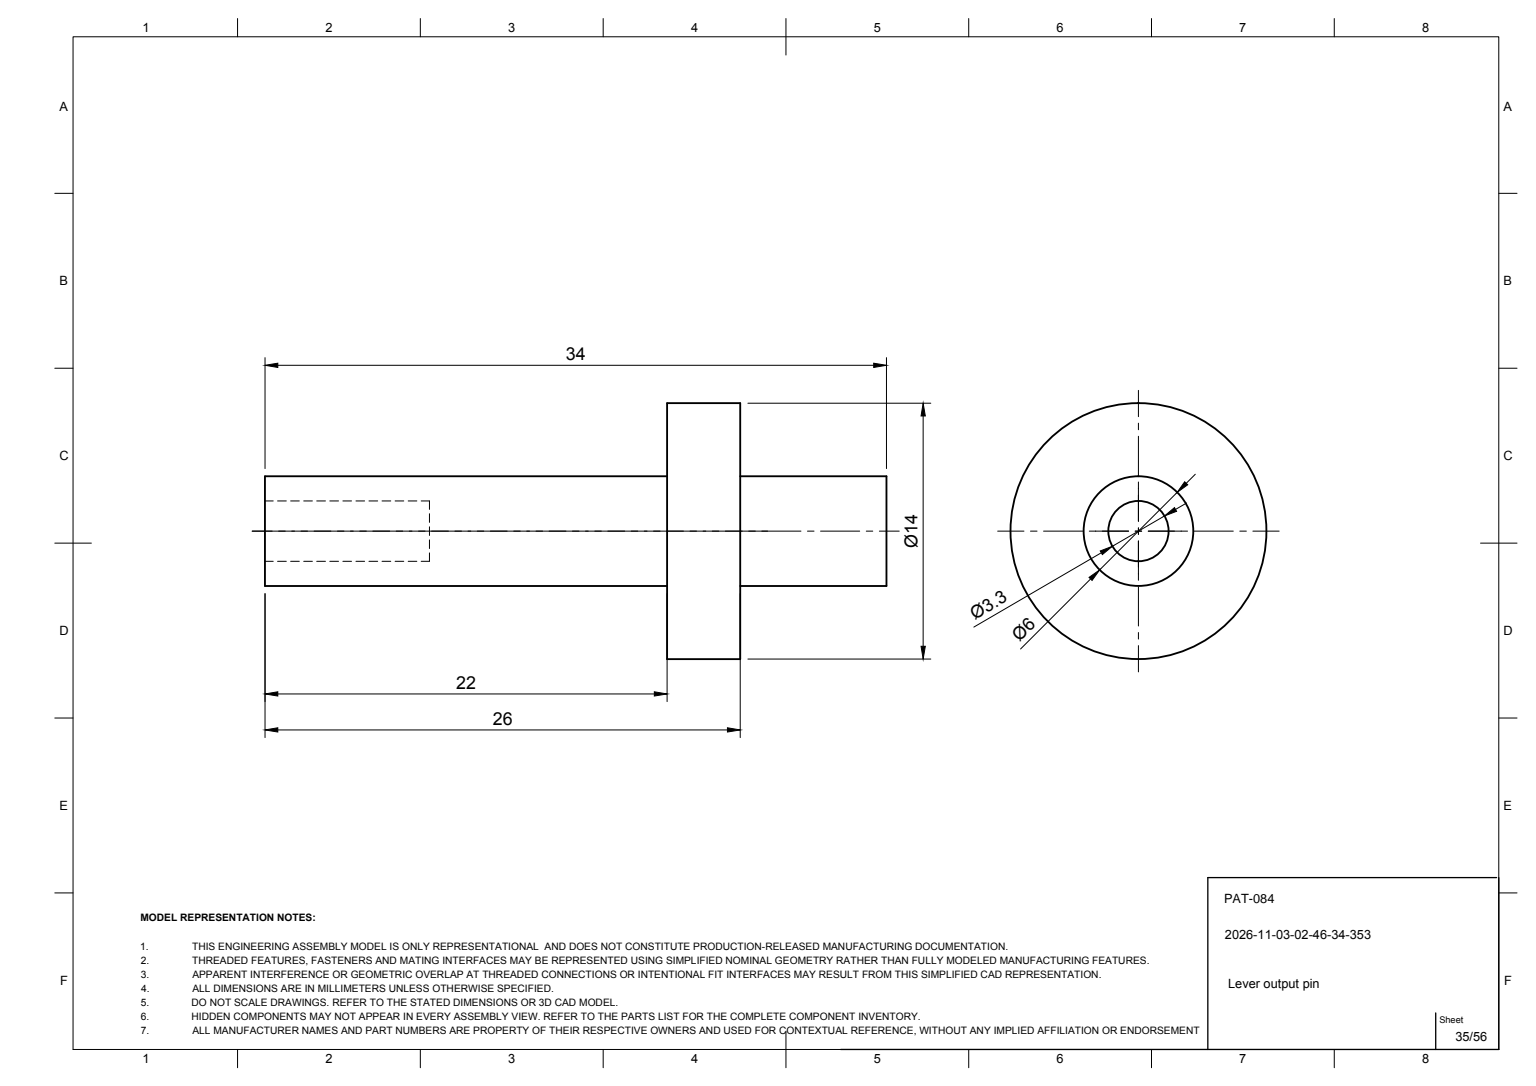
ISO-10303-21;
HEADER;
/* Generated by software containing ST-Developer
 * from STEP Tools, Inc. (www.steptools.com) 
 */

FILE_DESCRIPTION(
/* description */ ('Quick-return (Whitworth) mechanism'),
/* implementation_level */ '2;1');

FILE_NAME(
/* name */ 'Lever output pin.step',
/* time_stamp */ '2026-10-28T03:25:57-07:00',
/* author */ (''),
/* organization */ (''),
/* preprocessor_version */ 'ST-DEVELOPER v20.2',
/* originating_system */ 'Autodesk Translation Framework v15.17.0.0',
/* authorisation */ '');

FILE_SCHEMA (('AUTOMOTIVE_DESIGN { 1 0 10303 214 3 1 1 }'));
ENDSEC;

DATA;
#10=MECHANICAL_DESIGN_GEOMETRIC_PRESENTATION_REPRESENTATION('',(#523),#14878);
#427=SHAPE_REPRESENTATION_RELATIONSHIP('SRR','None',#15098,#471);
#471=ADVANCED_BREP_SHAPE_REPRESENTATION('',(#574),#14855);
#523=STYLED_ITEM('',(#15406),#574);
#574=MANIFOLD_SOLID_BREP('Body1',#7878);
#737=FACE_BOUND('',#1959,.T.);
#738=FACE_BOUND('',#1961,.T.);
#739=FACE_BOUND('',#1966,.T.);
#928=PLANE('',#9034);
#929=PLANE('',#9035);
#930=PLANE('',#9038);
#931=PLANE('',#9046);
#932=PLANE('',#9047);
#1344=FACE_OUTER_BOUND('',#1956,.T.);
#1345=FACE_OUTER_BOUND('',#1957,.T.);
#1346=FACE_OUTER_BOUND('',#1958,.T.);
#1347=FACE_OUTER_BOUND('',#1960,.T.);
#1348=FACE_OUTER_BOUND('',#1962,.T.);
#1349=FACE_OUTER_BOUND('',#1963,.T.);
#1350=FACE_OUTER_BOUND('',#1964,.T.);
#1351=FACE_OUTER_BOUND('',#1965,.T.);
#1352=FACE_OUTER_BOUND('',#1967,.T.);
#1956=EDGE_LOOP('',(#6492,#6493,#6494,#6495));
#1957=EDGE_LOOP('',(#6496));
#1958=EDGE_LOOP('',(#6497));
#1959=EDGE_LOOP('',(#6498));
#1960=EDGE_LOOP('',(#6499));
#1961=EDGE_LOOP('',(#6500));
#1962=EDGE_LOOP('',(#6501,#6502,#6503,#6504));
#1963=EDGE_LOOP('',(#6505,#6506,#6507,#6508));
#1964=EDGE_LOOP('',(#6509,#6510,#6511,#6512));
#1965=EDGE_LOOP('',(#6513));
#1966=EDGE_LOOP('',(#6514));
#1967=EDGE_LOOP('',(#6515));
#2435=LINE('',#13914,#2958);
#2436=LINE('',#13928,#2959);
#2437=LINE('',#13931,#2960);
#2438=LINE('',#13936,#2961);
#2958=VECTOR('',#10960,0.165);
#2959=VECTOR('',#10979,0.7);
#2960=VECTOR('',#10982,0.3);
#2961=VECTOR('',#10989,0.3);
#3530=CIRCLE('',#9032,0.165);
#3531=CIRCLE('',#9033,0.165);
#3532=CIRCLE('',#9036,0.7);
#3533=CIRCLE('',#9037,0.3);
#3534=CIRCLE('',#9039,0.7);
#3535=CIRCLE('',#9040,0.3);
#3536=CIRCLE('',#9043,0.3);
#3537=CIRCLE('',#9045,0.3);
#4051=VERTEX_POINT('',#13911);
#4052=VERTEX_POINT('',#13913);
#4053=VERTEX_POINT('',#13918);
#4054=VERTEX_POINT('',#13920);
#4055=VERTEX_POINT('',#13923);
#4056=VERTEX_POINT('',#13925);
#4057=VERTEX_POINT('',#13930);
#4058=VERTEX_POINT('',#13934);
#4903=EDGE_CURVE('',#4051,#4051,#3530,.T.);
#4904=EDGE_CURVE('',#4051,#4052,#2435,.T.);
#4905=EDGE_CURVE('',#4052,#4052,#3531,.T.);
#4906=EDGE_CURVE('',#4053,#4053,#3532,.T.);
#4907=EDGE_CURVE('',#4054,#4054,#3533,.T.);
#4908=EDGE_CURVE('',#4055,#4055,#3534,.T.);
#4909=EDGE_CURVE('',#4056,#4056,#3535,.T.);
#4910=EDGE_CURVE('',#4053,#4055,#2436,.T.);
#4911=EDGE_CURVE('',#4056,#4057,#2437,.T.);
#4912=EDGE_CURVE('',#4057,#4057,#3536,.T.);
#4913=EDGE_CURVE('',#4058,#4058,#3537,.T.);
#4914=EDGE_CURVE('',#4058,#4054,#2438,.T.);
#6492=ORIENTED_EDGE('',*,*,#4903,.F.);
#6493=ORIENTED_EDGE('',*,*,#4904,.T.);
#6494=ORIENTED_EDGE('',*,*,#4905,.F.);
#6495=ORIENTED_EDGE('',*,*,#4904,.F.);
#6496=ORIENTED_EDGE('',*,*,#4903,.T.);
#6497=ORIENTED_EDGE('',*,*,#4906,.T.);
#6498=ORIENTED_EDGE('',*,*,#4907,.F.);
#6499=ORIENTED_EDGE('',*,*,#4908,.F.);
#6500=ORIENTED_EDGE('',*,*,#4909,.F.);
#6501=ORIENTED_EDGE('',*,*,#4906,.F.);
#6502=ORIENTED_EDGE('',*,*,#4910,.T.);
#6503=ORIENTED_EDGE('',*,*,#4908,.T.);
#6504=ORIENTED_EDGE('',*,*,#4910,.F.);
#6505=ORIENTED_EDGE('',*,*,#4909,.T.);
#6506=ORIENTED_EDGE('',*,*,#4911,.T.);
#6507=ORIENTED_EDGE('',*,*,#4912,.T.);
#6508=ORIENTED_EDGE('',*,*,#4911,.F.);
#6509=ORIENTED_EDGE('',*,*,#4913,.F.);
#6510=ORIENTED_EDGE('',*,*,#4914,.T.);
#6511=ORIENTED_EDGE('',*,*,#4907,.T.);
#6512=ORIENTED_EDGE('',*,*,#4914,.F.);
#6513=ORIENTED_EDGE('',*,*,#4913,.T.);
#6514=ORIENTED_EDGE('',*,*,#4905,.T.);
#6515=ORIENTED_EDGE('',*,*,#4912,.F.);
#7335=CYLINDRICAL_SURFACE('',#9031,0.165);
#7336=CYLINDRICAL_SURFACE('',#9041,0.7);
#7337=CYLINDRICAL_SURFACE('',#9042,0.3);
#7338=CYLINDRICAL_SURFACE('',#9044,0.3);
#7675=ADVANCED_FACE('',(#1344),#7335,.F.);
#7676=ADVANCED_FACE('',(#1345),#928,.T.);
#7677=ADVANCED_FACE('',(#1346,#737),#929,.T.);
#7678=ADVANCED_FACE('',(#1347,#738),#930,.F.);
#7679=ADVANCED_FACE('',(#1348),#7336,.T.);
#7680=ADVANCED_FACE('',(#1349),#7337,.T.);
#7681=ADVANCED_FACE('',(#1350),#7338,.T.);
#7682=ADVANCED_FACE('',(#1351,#739),#931,.T.);
#7683=ADVANCED_FACE('',(#1352),#932,.F.);
#7878=CLOSED_SHELL('',(#7675,#7676,#7677,#7678,#7679,#7680,#7681,#7682,
#7683));
#9030=AXIS2_PLACEMENT_3D('',#13909,#10954,#10955);
#9031=AXIS2_PLACEMENT_3D('',#13910,#10956,#10957);
#9032=AXIS2_PLACEMENT_3D('',#13912,#10958,#10959);
#9033=AXIS2_PLACEMENT_3D('',#13915,#10961,#10962);
#9034=AXIS2_PLACEMENT_3D('',#13916,#10963,#10964);
#9035=AXIS2_PLACEMENT_3D('',#13917,#10965,#10966);
#9036=AXIS2_PLACEMENT_3D('',#13919,#10967,#10968);
#9037=AXIS2_PLACEMENT_3D('',#13921,#10969,#10970);
#9038=AXIS2_PLACEMENT_3D('',#13922,#10971,#10972);
#9039=AXIS2_PLACEMENT_3D('',#13924,#10973,#10974);
#9040=AXIS2_PLACEMENT_3D('',#13926,#10975,#10976);
#9041=AXIS2_PLACEMENT_3D('',#13927,#10977,#10978);
#9042=AXIS2_PLACEMENT_3D('',#13929,#10980,#10981);
#9043=AXIS2_PLACEMENT_3D('',#13932,#10983,#10984);
#9044=AXIS2_PLACEMENT_3D('',#13933,#10985,#10986);
#9045=AXIS2_PLACEMENT_3D('',#13935,#10987,#10988);
#9046=AXIS2_PLACEMENT_3D('',#13937,#10990,#10991);
#9047=AXIS2_PLACEMENT_3D('',#13938,#10992,#10993);
#10954=DIRECTION('axis',(0.,0.,1.));
#10955=DIRECTION('refdir',(1.,0.,0.));
#10956=DIRECTION('center_axis',(0.,0.,1.));
#10957=DIRECTION('ref_axis',(1.,0.,0.));
#10958=DIRECTION('center_axis',(0.,0.,1.));
#10959=DIRECTION('ref_axis',(1.,0.,0.));
#10960=DIRECTION('',(0.,0.,1.));
#10961=DIRECTION('center_axis',(0.,0.,-1.));
#10962=DIRECTION('ref_axis',(1.,0.,0.));
#10963=DIRECTION('center_axis',(0.,0.,1.));
#10964=DIRECTION('ref_axis',(1.,0.,0.));
#10965=DIRECTION('center_axis',(0.,0.,1.));
#10966=DIRECTION('ref_axis',(1.,0.,0.));
#10967=DIRECTION('center_axis',(0.,0.,1.));
#10968=DIRECTION('ref_axis',(1.,0.,0.));
#10969=DIRECTION('center_axis',(0.,0.,1.));
#10970=DIRECTION('ref_axis',(1.,0.,0.));
#10971=DIRECTION('center_axis',(0.,0.,1.));
#10972=DIRECTION('ref_axis',(1.,0.,0.));
#10973=DIRECTION('center_axis',(0.,0.,1.));
#10974=DIRECTION('ref_axis',(1.,0.,0.));
#10975=DIRECTION('center_axis',(0.,0.,-1.));
#10976=DIRECTION('ref_axis',(1.,0.,0.));
#10977=DIRECTION('center_axis',(0.,0.,1.));
#10978=DIRECTION('ref_axis',(1.,0.,0.));
#10979=DIRECTION('',(0.,0.,-1.));
#10980=DIRECTION('center_axis',(0.,0.,1.));
#10981=DIRECTION('ref_axis',(1.,0.,0.));
#10982=DIRECTION('',(0.,0.,-1.));
#10983=DIRECTION('center_axis',(0.,0.,1.));
#10984=DIRECTION('ref_axis',(1.,0.,0.));
#10985=DIRECTION('center_axis',(0.,0.,1.));
#10986=DIRECTION('ref_axis',(1.,0.,0.));
#10987=DIRECTION('center_axis',(0.,0.,1.));
#10988=DIRECTION('ref_axis',(1.,0.,0.));
#10989=DIRECTION('',(0.,0.,-1.));
#10990=DIRECTION('center_axis',(0.,0.,1.));
#10991=DIRECTION('ref_axis',(1.,0.,0.));
#10992=DIRECTION('center_axis',(0.,0.,1.));
#10993=DIRECTION('ref_axis',(1.,0.,0.));
#13909=CARTESIAN_POINT('',(0.,0.,0.));
#13910=CARTESIAN_POINT('Origin',(0.,12.,8.9));
#13911=CARTESIAN_POINT('',(-0.165,12.,8.9));
#13912=CARTESIAN_POINT('Origin',(0.,12.,8.9));
#13913=CARTESIAN_POINT('',(-0.165,12.,9.8));
#13914=CARTESIAN_POINT('',(-0.165,12.,8.9));
#13915=CARTESIAN_POINT('Origin',(0.,12.,9.8));
#13916=CARTESIAN_POINT('Origin',(0.,12.,8.9));
#13917=CARTESIAN_POINT('Origin',(0.,12.,7.6));
#13918=CARTESIAN_POINT('',(-0.7,12.,7.6));
#13919=CARTESIAN_POINT('Origin',(0.,12.,7.6));
#13920=CARTESIAN_POINT('',(-0.3,12.,7.6));
#13921=CARTESIAN_POINT('Origin',(0.,12.,7.6));
#13922=CARTESIAN_POINT('Origin',(0.,12.,7.2));
#13923=CARTESIAN_POINT('',(-0.7,12.,7.2));
#13924=CARTESIAN_POINT('Origin',(0.,12.,7.2));
#13925=CARTESIAN_POINT('',(-0.3,12.,7.2));
#13926=CARTESIAN_POINT('Origin',(0.,12.,7.2));
#13927=CARTESIAN_POINT('Origin',(0.,12.,7.2));
#13928=CARTESIAN_POINT('',(-0.7,12.,7.2));
#13929=CARTESIAN_POINT('Origin',(0.,12.,6.4));
#13930=CARTESIAN_POINT('',(-0.3,12.,6.4));
#13931=CARTESIAN_POINT('',(-0.3,12.,6.4));
#13932=CARTESIAN_POINT('Origin',(0.,12.,6.4));
#13933=CARTESIAN_POINT('Origin',(0.,12.,6.4));
#13934=CARTESIAN_POINT('',(-0.3,12.,9.8));
#13935=CARTESIAN_POINT('Origin',(0.,12.,9.8));
#13936=CARTESIAN_POINT('',(-0.3,12.,6.4));
#13937=CARTESIAN_POINT('Origin',(0.,12.,9.8));
#13938=CARTESIAN_POINT('Origin',(0.,12.,6.4));
#14801=UNCERTAINTY_MEASURE_WITH_UNIT(LENGTH_MEASURE(0.001),#14879,
'DISTANCE_ACCURACY_VALUE',
'Maximum model space distance between geometric entities at asserted c
onnectivities');
#14824=UNCERTAINTY_MEASURE_WITH_UNIT(LENGTH_MEASURE(0.001),#14879,
'DISTANCE_ACCURACY_VALUE',
'Maximum model space distance between geometric entities at asserted c
onnectivities');
#14855=(
GEOMETRIC_REPRESENTATION_CONTEXT(3)
GLOBAL_UNCERTAINTY_ASSIGNED_CONTEXT((#14801))
GLOBAL_UNIT_ASSIGNED_CONTEXT((#14879,#14881,#14882))
REPRESENTATION_CONTEXT('','3D')
);
#14878=(
GEOMETRIC_REPRESENTATION_CONTEXT(3)
GLOBAL_UNCERTAINTY_ASSIGNED_CONTEXT((#14824))
GLOBAL_UNIT_ASSIGNED_CONTEXT((#14879,#14881,#14882))
REPRESENTATION_CONTEXT('','3D')
);
#14879=(
LENGTH_UNIT()
NAMED_UNIT(*)
SI_UNIT(.CENTI.,.METRE.)
);
#14881=(
NAMED_UNIT(*)
PLANE_ANGLE_UNIT()
SI_UNIT($,.RADIAN.)
);
#14882=(
NAMED_UNIT(*)
SI_UNIT($,.STERADIAN.)
SOLID_ANGLE_UNIT()
);
#14913=SHAPE_DEFINITION_REPRESENTATION(#14971,#15098);
#14971=PRODUCT_DEFINITION_SHAPE('',$,#15152);
#15098=SHAPE_REPRESENTATION('',(#9030),#14855);
#15121=PRODUCT_DEFINITION_CONTEXT('part definition',#15282,'design');
#15152=PRODUCT_DEFINITION('Lever output pin','Lever output pin',#15205,
#15121);
#15205=PRODUCT_DEFINITION_FORMATION('',$,#15314);
#15282=APPLICATION_CONTEXT(
'Core Data for Automotive Mechanical Design Process');
#15283=PRODUCT_CONTEXT('part definition',#15282,'mechanical');
#15314=PRODUCT('Lever output pin','Lever output pin','Lever output pin',
(#15283));
#15400=COLOUR_RGB('Grey',0.48,0.52,0.57);
#15401=FILL_AREA_STYLE_COLOUR('',#15400);
#15402=FILL_AREA_STYLE('',(#15401));
#15403=SURFACE_STYLE_FILL_AREA(#15402);
#15404=SURFACE_SIDE_STYLE('',(#15403));
#15405=SURFACE_STYLE_USAGE(.BOTH.,#15404);
#15406=PRESENTATION_STYLE_ASSIGNMENT((#15405));
ENDSEC;
END-ISO-10303-21;
